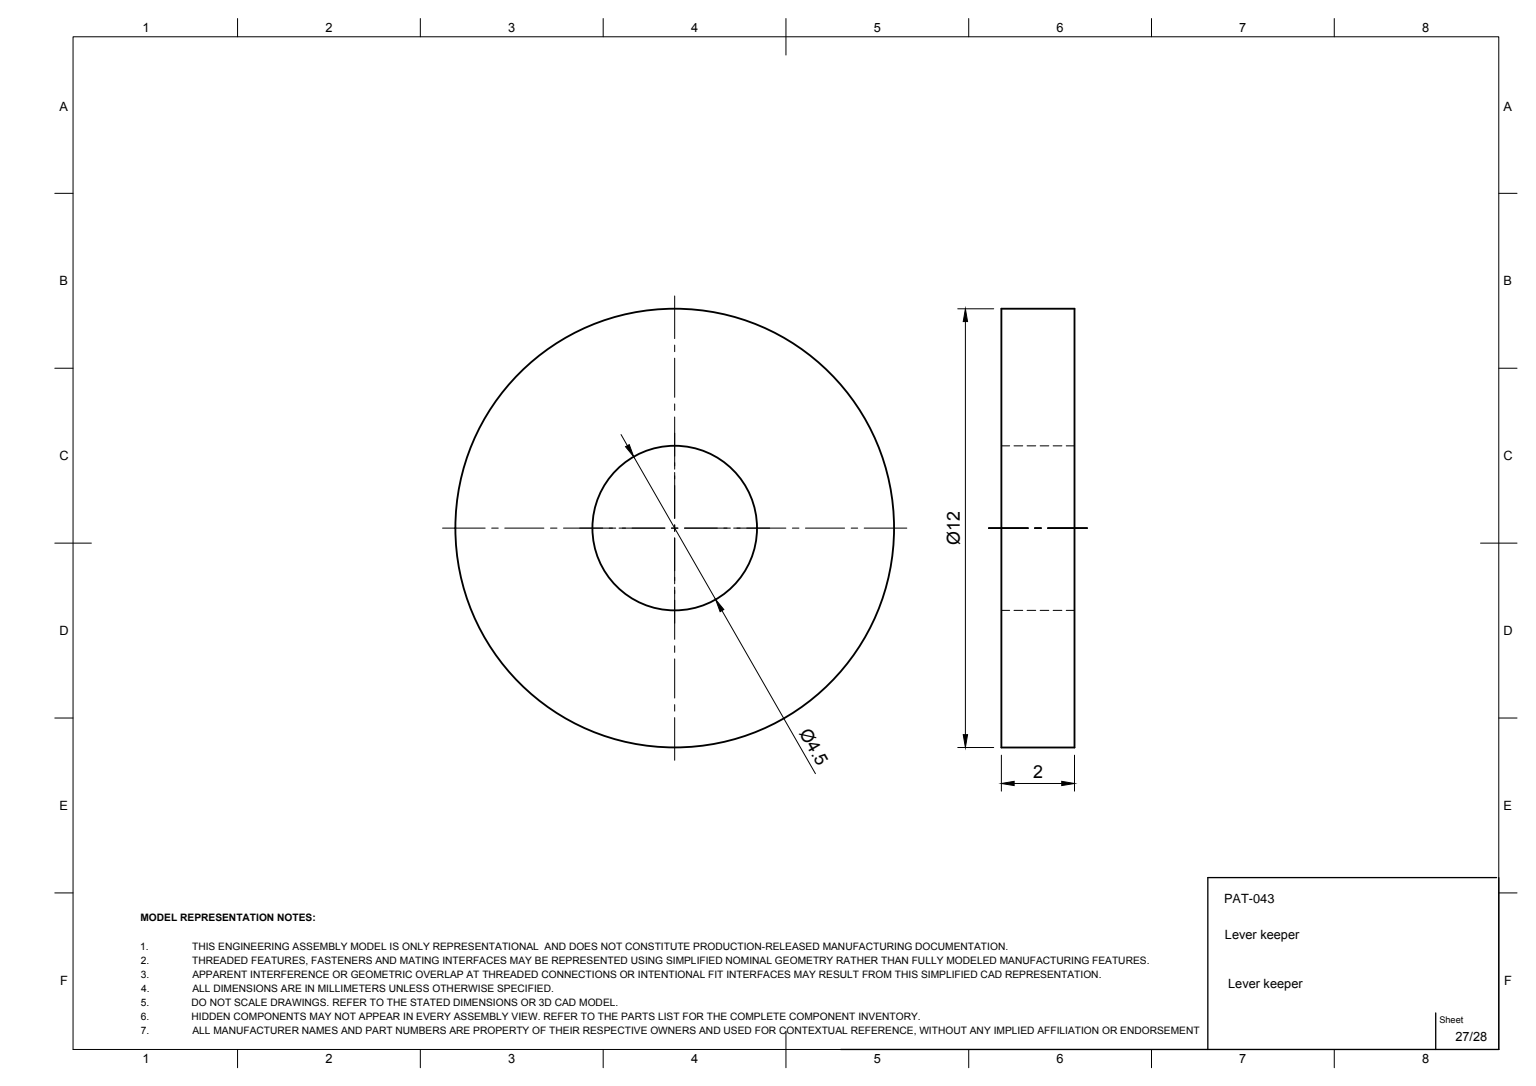
ISO-10303-21;
HEADER;
/* Generated by software containing ST-Developer
 * from STEP Tools, Inc. (www.steptools.com) 
 */

FILE_DESCRIPTION(
/* description */ ('Four-valve pipe header'),
/* implementation_level */ '2;1');

FILE_NAME(
/* name */ 'Lever keeper.step',
/* time_stamp */ '2026-10-29T16:56:19-07:00',
/* author */ (''),
/* organization */ (''),
/* preprocessor_version */ 'ST-DEVELOPER v20.2',
/* originating_system */ 'Autodesk Translation Framework v15.17.0.0',
/* authorisation */ '');

FILE_SCHEMA (('AUTOMOTIVE_DESIGN { 1 0 10303 214 3 1 1 }'));
ENDSEC;

DATA;
#10=MECHANICAL_DESIGN_GEOMETRIC_PRESENTATION_REPRESENTATION('',(#356),#10119);
#304=SHAPE_REPRESENTATION_RELATIONSHIP('SRR','None',#10267,#330);
#330=ADVANCED_BREP_SHAPE_REPRESENTATION('',(#380),#10116);
#356=STYLED_ITEM('',(#10463),#380);
#380=MANIFOLD_SOLID_BREP('Body1',#5604);
#532=FACE_BOUND('',#1494,.T.);
#533=FACE_BOUND('',#1496,.T.);
#728=PLANE('',#6480);
#729=PLANE('',#6481);
#1053=FACE_OUTER_BOUND('',#1491,.T.);
#1054=FACE_OUTER_BOUND('',#1492,.T.);
#1055=FACE_OUTER_BOUND('',#1493,.T.);
#1056=FACE_OUTER_BOUND('',#1495,.T.);
#1491=EDGE_LOOP('',(#5053,#5054,#5055,#5056));
#1492=EDGE_LOOP('',(#5057,#5058,#5059,#5060));
#1493=EDGE_LOOP('',(#5061));
#1494=EDGE_LOOP('',(#5062));
#1495=EDGE_LOOP('',(#5063));
#1496=EDGE_LOOP('',(#5064));
#1901=LINE('',#9899,#2319);
#1902=LINE('',#9905,#2320);
#2319=VECTOR('',#8112,0.225);
#2320=VECTOR('',#8119,0.6);
#2569=CIRCLE('',#6475,0.225);
#2570=CIRCLE('',#6476,0.225);
#2571=CIRCLE('',#6478,0.6);
#2572=CIRCLE('',#6479,0.6);
#3006=VERTEX_POINT('',#9896);
#3007=VERTEX_POINT('',#9898);
#3008=VERTEX_POINT('',#9902);
#3009=VERTEX_POINT('',#9904);
#3693=EDGE_CURVE('',#3006,#3006,#2569,.T.);
#3694=EDGE_CURVE('',#3006,#3007,#1901,.T.);
#3695=EDGE_CURVE('',#3007,#3007,#2570,.T.);
#3696=EDGE_CURVE('',#3008,#3008,#2571,.T.);
#3697=EDGE_CURVE('',#3008,#3009,#1902,.T.);
#3698=EDGE_CURVE('',#3009,#3009,#2572,.T.);
#5053=ORIENTED_EDGE('',*,*,#3693,.F.);
#5054=ORIENTED_EDGE('',*,*,#3694,.T.);
#5055=ORIENTED_EDGE('',*,*,#3695,.T.);
#5056=ORIENTED_EDGE('',*,*,#3694,.F.);
#5057=ORIENTED_EDGE('',*,*,#3696,.F.);
#5058=ORIENTED_EDGE('',*,*,#3697,.T.);
#5059=ORIENTED_EDGE('',*,*,#3698,.T.);
#5060=ORIENTED_EDGE('',*,*,#3697,.F.);
#5061=ORIENTED_EDGE('',*,*,#3696,.T.);
#5062=ORIENTED_EDGE('',*,*,#3693,.T.);
#5063=ORIENTED_EDGE('',*,*,#3698,.F.);
#5064=ORIENTED_EDGE('',*,*,#3695,.F.);
#5243=CYLINDRICAL_SURFACE('',#6474,0.225);
#5244=CYLINDRICAL_SURFACE('',#6477,0.6);
#5553=ADVANCED_FACE('',(#1053),#5243,.F.);
#5554=ADVANCED_FACE('',(#1054),#5244,.T.);
#5555=ADVANCED_FACE('',(#1055,#532),#728,.T.);
#5556=ADVANCED_FACE('',(#1056,#533),#729,.F.);
#5604=CLOSED_SHELL('',(#5553,#5554,#5555,#5556));
#6473=AXIS2_PLACEMENT_3D('',#9894,#8106,#8107);
#6474=AXIS2_PLACEMENT_3D('',#9895,#8108,#8109);
#6475=AXIS2_PLACEMENT_3D('',#9897,#8110,#8111);
#6476=AXIS2_PLACEMENT_3D('',#9900,#8113,#8114);
#6477=AXIS2_PLACEMENT_3D('',#9901,#8115,#8116);
#6478=AXIS2_PLACEMENT_3D('',#9903,#8117,#8118);
#6479=AXIS2_PLACEMENT_3D('',#9906,#8120,#8121);
#6480=AXIS2_PLACEMENT_3D('',#9907,#8122,#8123);
#6481=AXIS2_PLACEMENT_3D('',#9908,#8124,#8125);
#8106=DIRECTION('axis',(0.,0.,1.));
#8107=DIRECTION('refdir',(1.,0.,0.));
#8108=DIRECTION('center_axis',(0.,0.,1.));
#8109=DIRECTION('ref_axis',(1.,0.,0.));
#8110=DIRECTION('center_axis',(0.,0.,-1.));
#8111=DIRECTION('ref_axis',(1.,0.,0.));
#8112=DIRECTION('',(0.,0.,-1.));
#8113=DIRECTION('center_axis',(0.,0.,-1.));
#8114=DIRECTION('ref_axis',(1.,0.,0.));
#8115=DIRECTION('center_axis',(0.,0.,1.));
#8116=DIRECTION('ref_axis',(1.,0.,0.));
#8117=DIRECTION('center_axis',(0.,0.,1.));
#8118=DIRECTION('ref_axis',(1.,0.,0.));
#8119=DIRECTION('',(0.,0.,-1.));
#8120=DIRECTION('center_axis',(0.,0.,1.));
#8121=DIRECTION('ref_axis',(1.,0.,0.));
#8122=DIRECTION('center_axis',(0.,0.,1.));
#8123=DIRECTION('ref_axis',(1.,0.,0.));
#8124=DIRECTION('center_axis',(0.,0.,1.));
#8125=DIRECTION('ref_axis',(1.,0.,0.));
#9894=CARTESIAN_POINT('',(0.,0.,0.));
#9895=CARTESIAN_POINT('Origin',(0.,0.,9.4));
#9896=CARTESIAN_POINT('',(-0.225,-2.75545529808154E-17,9.6));
#9897=CARTESIAN_POINT('Origin',(0.,0.,9.6));
#9898=CARTESIAN_POINT('',(-0.225,-2.75545529808154E-17,9.4));
#9899=CARTESIAN_POINT('',(-0.225,-2.75545529808154E-17,9.4));
#9900=CARTESIAN_POINT('Origin',(0.,0.,9.4));
#9901=CARTESIAN_POINT('Origin',(0.,0.,9.4));
#9902=CARTESIAN_POINT('',(-0.6,-7.34788079488412E-17,9.6));
#9903=CARTESIAN_POINT('Origin',(0.,0.,9.6));
#9904=CARTESIAN_POINT('',(-0.6,-7.34788079488412E-17,9.4));
#9905=CARTESIAN_POINT('',(-0.6,-7.34788079488412E-17,9.4));
#9906=CARTESIAN_POINT('Origin',(0.,0.,9.4));
#9907=CARTESIAN_POINT('Origin',(0.,0.,9.6));
#9908=CARTESIAN_POINT('Origin',(0.,0.,9.4));
#10085=UNCERTAINTY_MEASURE_WITH_UNIT(LENGTH_MEASURE(0.001),#10120,
'DISTANCE_ACCURACY_VALUE',
'Maximum model space distance between geometric entities at asserted c
onnectivities');
#10088=UNCERTAINTY_MEASURE_WITH_UNIT(LENGTH_MEASURE(0.001),#10120,
'DISTANCE_ACCURACY_VALUE',
'Maximum model space distance between geometric entities at asserted c
onnectivities');
#10116=(
GEOMETRIC_REPRESENTATION_CONTEXT(3)
GLOBAL_UNCERTAINTY_ASSIGNED_CONTEXT((#10085))
GLOBAL_UNIT_ASSIGNED_CONTEXT((#10120,#10122,#10123))
REPRESENTATION_CONTEXT('','3D')
);
#10119=(
GEOMETRIC_REPRESENTATION_CONTEXT(3)
GLOBAL_UNCERTAINTY_ASSIGNED_CONTEXT((#10088))
GLOBAL_UNIT_ASSIGNED_CONTEXT((#10120,#10122,#10123))
REPRESENTATION_CONTEXT('','3D')
);
#10120=(
LENGTH_UNIT()
NAMED_UNIT(*)
SI_UNIT(.CENTI.,.METRE.)
);
#10122=(
NAMED_UNIT(*)
PLANE_ANGLE_UNIT()
SI_UNIT($,.RADIAN.)
);
#10123=(
NAMED_UNIT(*)
SI_UNIT($,.STERADIAN.)
SOLID_ANGLE_UNIT()
);
#10151=SHAPE_DEFINITION_REPRESENTATION(#10181,#10267);
#10181=PRODUCT_DEFINITION_SHAPE('',$,#10298);
#10267=SHAPE_REPRESENTATION('',(#6473),#10116);
#10270=PRODUCT_DEFINITION_CONTEXT('part definition',#10362,'design');
#10298=PRODUCT_DEFINITION('Lever keeper','Lever keeper',#10328,#10270);
#10328=PRODUCT_DEFINITION_FORMATION('',$,#10391);
#10362=APPLICATION_CONTEXT(
'Core Data for Automotive Mechanical Design Process');
#10363=PRODUCT_CONTEXT('part definition',#10362,'mechanical');
#10391=PRODUCT('Lever keeper','Lever keeper','Lever keeper',(#10363));
#10457=COLOUR_RGB('Sky Blue',0.24,0.69,0.87);
#10458=FILL_AREA_STYLE_COLOUR('',#10457);
#10459=FILL_AREA_STYLE('',(#10458));
#10460=SURFACE_STYLE_FILL_AREA(#10459);
#10461=SURFACE_SIDE_STYLE('',(#10460));
#10462=SURFACE_STYLE_USAGE(.BOTH.,#10461);
#10463=PRESENTATION_STYLE_ASSIGNMENT((#10462));
ENDSEC;
END-ISO-10303-21;
